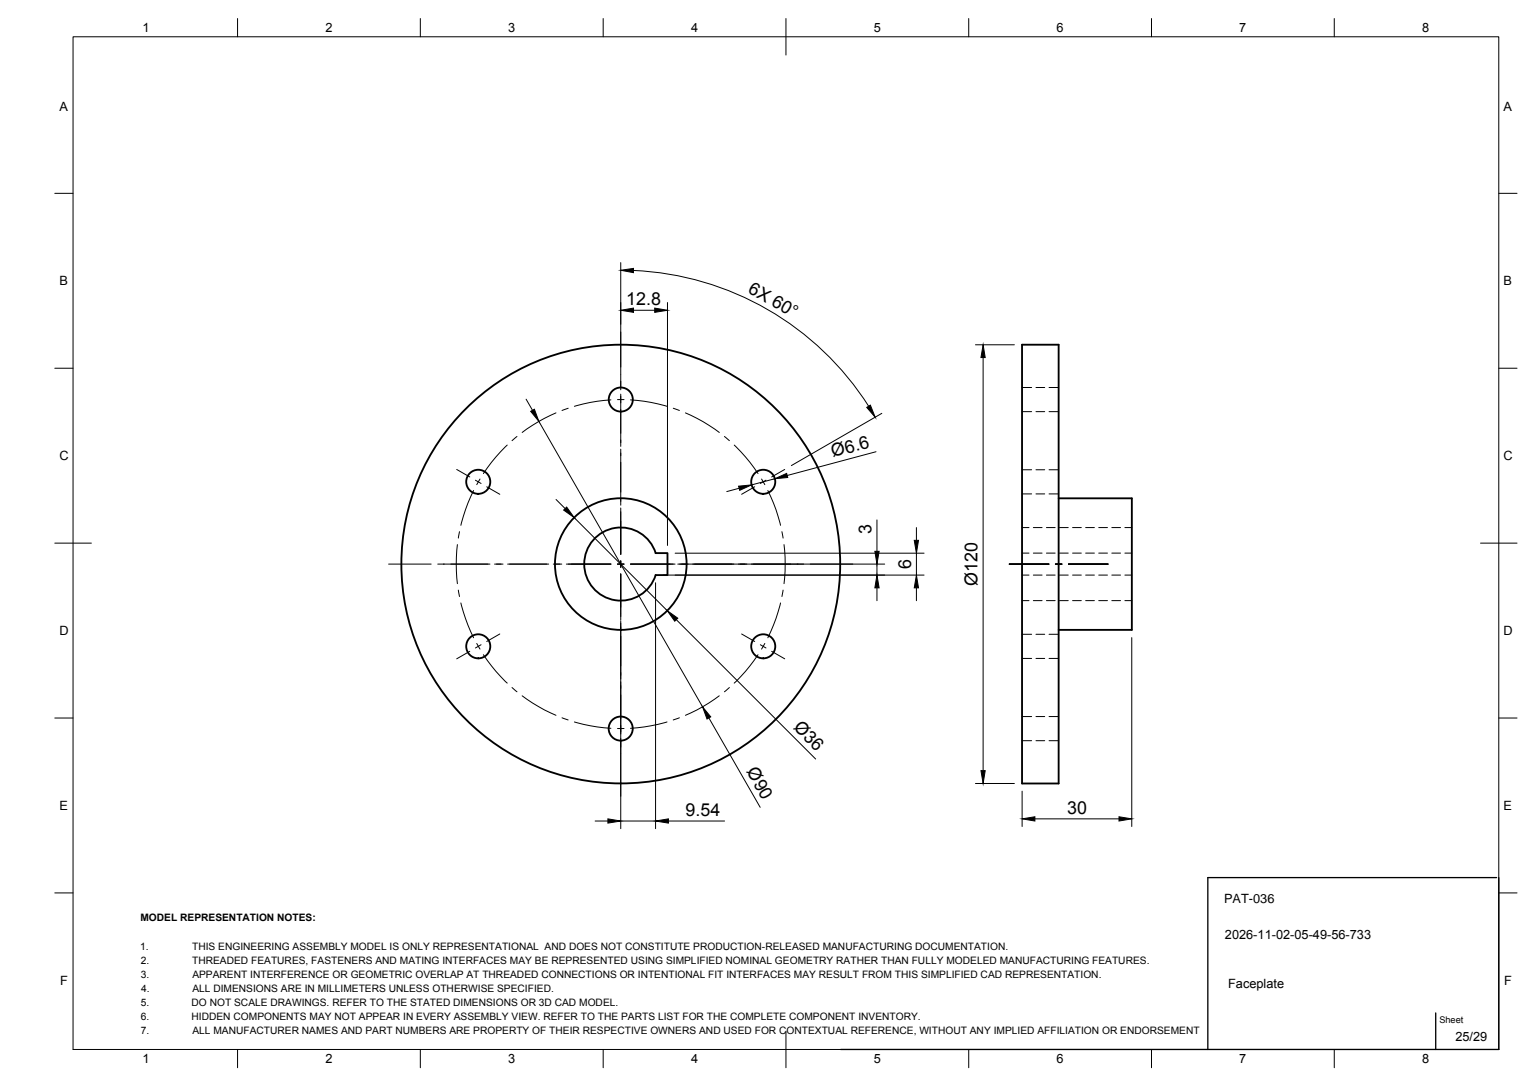
ISO-10303-21;
HEADER;
/* Generated by software containing ST-Developer
 * from STEP Tools, Inc. (www.steptools.com) 
 */

FILE_DESCRIPTION(
/* description */ ('Flange-mounted spindle'),
/* implementation_level */ '2;1');

FILE_NAME(
/* name */ 'Faceplate.step',
/* time_stamp */ '2026-10-27T10:49:51-07:00',
/* author */ (''),
/* organization */ (''),
/* preprocessor_version */ 'ST-DEVELOPER v20.2',
/* originating_system */ 'Autodesk Translation Framework v15.17.0.0',
/* authorisation */ '');

FILE_SCHEMA (('AUTOMOTIVE_DESIGN { 1 0 10303 214 3 1 1 }'));
ENDSEC;

DATA;
#10=MECHANICAL_DESIGN_GEOMETRIC_PRESENTATION_REPRESENTATION('',(#357),#11764);
#302=SHAPE_REPRESENTATION_RELATIONSHIP('SRR','None',#11900,#329);
#329=ADVANCED_BREP_SHAPE_REPRESENTATION('',(#383),#11755);
#357=STYLED_ITEM('',(#12085),#383);
#383=MANIFOLD_SOLID_BREP('Body1',#6151);
#471=FACE_BOUND('',#1269,.T.);
#472=FACE_BOUND('',#1270,.T.);
#473=FACE_BOUND('',#1271,.T.);
#474=FACE_BOUND('',#1272,.T.);
#475=FACE_BOUND('',#1273,.T.);
#476=FACE_BOUND('',#1274,.T.);
#477=FACE_BOUND('',#1275,.T.);
#478=FACE_BOUND('',#1284,.T.);
#479=FACE_BOUND('',#1285,.T.);
#480=FACE_BOUND('',#1286,.T.);
#481=FACE_BOUND('',#1287,.T.);
#482=FACE_BOUND('',#1288,.T.);
#483=FACE_BOUND('',#1289,.T.);
#484=FACE_BOUND('',#1290,.T.);
#485=FACE_BOUND('',#1294,.T.);
#608=PLANE('',#6765);
#609=PLANE('',#6766);
#610=PLANE('',#6767);
#611=PLANE('',#6768);
#612=PLANE('',#6791);
#613=PLANE('',#6797);
#840=FACE_OUTER_BOUND('',#1265,.T.);
#841=FACE_OUTER_BOUND('',#1266,.T.);
#842=FACE_OUTER_BOUND('',#1267,.T.);
#843=FACE_OUTER_BOUND('',#1268,.T.);
#844=FACE_OUTER_BOUND('',#1276,.T.);
#845=FACE_OUTER_BOUND('',#1277,.T.);
#846=FACE_OUTER_BOUND('',#1278,.T.);
#847=FACE_OUTER_BOUND('',#1279,.T.);
#848=FACE_OUTER_BOUND('',#1280,.T.);
#849=FACE_OUTER_BOUND('',#1281,.T.);
#850=FACE_OUTER_BOUND('',#1282,.T.);
#851=FACE_OUTER_BOUND('',#1283,.T.);
#852=FACE_OUTER_BOUND('',#1291,.T.);
#853=FACE_OUTER_BOUND('',#1292,.T.);
#854=FACE_OUTER_BOUND('',#1293,.T.);
#1265=EDGE_LOOP('',(#4699,#4700,#4701,#4702));
#1266=EDGE_LOOP('',(#4703,#4704,#4705,#4706));
#1267=EDGE_LOOP('',(#4707,#4708,#4709,#4710));
#1268=EDGE_LOOP('',(#4711));
#1269=EDGE_LOOP('',(#4712));
#1270=EDGE_LOOP('',(#4713));
#1271=EDGE_LOOP('',(#4714));
#1272=EDGE_LOOP('',(#4715));
#1273=EDGE_LOOP('',(#4716));
#1274=EDGE_LOOP('',(#4717));
#1275=EDGE_LOOP('',(#4718,#4719,#4720,#4721));
#1276=EDGE_LOOP('',(#4722,#4723,#4724,#4725));
#1277=EDGE_LOOP('',(#4726,#4727,#4728,#4729));
#1278=EDGE_LOOP('',(#4730,#4731,#4732,#4733));
#1279=EDGE_LOOP('',(#4734,#4735,#4736,#4737));
#1280=EDGE_LOOP('',(#4738,#4739,#4740,#4741));
#1281=EDGE_LOOP('',(#4742,#4743,#4744,#4745));
#1282=EDGE_LOOP('',(#4746,#4747,#4748,#4749));
#1283=EDGE_LOOP('',(#4750));
#1284=EDGE_LOOP('',(#4751));
#1285=EDGE_LOOP('',(#4752));
#1286=EDGE_LOOP('',(#4753));
#1287=EDGE_LOOP('',(#4754));
#1288=EDGE_LOOP('',(#4755));
#1289=EDGE_LOOP('',(#4756));
#1290=EDGE_LOOP('',(#4757));
#1291=EDGE_LOOP('',(#4758,#4759,#4760,#4761));
#1292=EDGE_LOOP('',(#4762,#4763,#4764,#4765));
#1293=EDGE_LOOP('',(#4766));
#1294=EDGE_LOOP('',(#4767,#4768,#4769,#4770));
#1679=LINE('',#10434,#2101);
#1680=LINE('',#10436,#2102);
#1681=LINE('',#10438,#2103);
#1682=LINE('',#10439,#2104);
#1683=LINE('',#10442,#2105);
#1684=LINE('',#10444,#2106);
#1685=LINE('',#10445,#2107);
#1686=LINE('',#10448,#2108);
#1687=LINE('',#10450,#2109);
#1688=LINE('',#10451,#2110);
#1689=LINE('',#10473,#2111);
#1690=LINE('',#10477,#2112);
#1691=LINE('',#10481,#2113);
#1692=LINE('',#10485,#2114);
#1693=LINE('',#10489,#2115);
#1694=LINE('',#10493,#2116);
#1695=LINE('',#10500,#2117);
#1696=LINE('',#10503,#2118);
#2101=VECTOR('',#8022,1.);
#2102=VECTOR('',#8023,1.);
#2103=VECTOR('',#8024,1.);
#2104=VECTOR('',#8025,1.);
#2105=VECTOR('',#8028,1.);
#2106=VECTOR('',#8029,1.);
#2107=VECTOR('',#8030,1.);
#2108=VECTOR('',#8033,1.);
#2109=VECTOR('',#8034,1.);
#2110=VECTOR('',#8035,1.);
#2111=VECTOR('',#8062,0.33);
#2112=VECTOR('',#8067,0.33);
#2113=VECTOR('',#8072,0.33);
#2114=VECTOR('',#8077,0.33);
#2115=VECTOR('',#8082,0.33);
#2116=VECTOR('',#8087,0.33);
#2117=VECTOR('',#8096,6.);
#2118=VECTOR('',#8099,1.8);
#2438=CIRCLE('',#6769,6.);
#2439=CIRCLE('',#6770,0.33);
#2440=CIRCLE('',#6771,0.33);
#2441=CIRCLE('',#6772,0.33);
#2442=CIRCLE('',#6773,0.33);
#2443=CIRCLE('',#6774,0.33);
#2444=CIRCLE('',#6775,0.33);
#2445=CIRCLE('',#6776,1.);
#2446=CIRCLE('',#6778,1.);
#2447=CIRCLE('',#6780,0.33);
#2448=CIRCLE('',#6782,0.33);
#2449=CIRCLE('',#6784,0.33);
#2450=CIRCLE('',#6786,0.33);
#2451=CIRCLE('',#6788,0.33);
#2452=CIRCLE('',#6790,0.33);
#2453=CIRCLE('',#6792,6.);
#2454=CIRCLE('',#6793,1.8);
#2455=CIRCLE('',#6796,1.8);
#2886=VERTEX_POINT('',#10432);
#2887=VERTEX_POINT('',#10433);
#2888=VERTEX_POINT('',#10435);
#2889=VERTEX_POINT('',#10437);
#2890=VERTEX_POINT('',#10441);
#2891=VERTEX_POINT('',#10443);
#2892=VERTEX_POINT('',#10447);
#2893=VERTEX_POINT('',#10449);
#2894=VERTEX_POINT('',#10453);
#2895=VERTEX_POINT('',#10455);
#2896=VERTEX_POINT('',#10457);
#2897=VERTEX_POINT('',#10459);
#2898=VERTEX_POINT('',#10461);
#2899=VERTEX_POINT('',#10463);
#2900=VERTEX_POINT('',#10465);
#2901=VERTEX_POINT('',#10471);
#2902=VERTEX_POINT('',#10475);
#2903=VERTEX_POINT('',#10479);
#2904=VERTEX_POINT('',#10483);
#2905=VERTEX_POINT('',#10487);
#2906=VERTEX_POINT('',#10491);
#2907=VERTEX_POINT('',#10495);
#2908=VERTEX_POINT('',#10497);
#2909=VERTEX_POINT('',#10502);
#3542=EDGE_CURVE('',#2886,#2887,#1679,.T.);
#3543=EDGE_CURVE('',#2886,#2888,#1680,.T.);
#3544=EDGE_CURVE('',#2889,#2888,#1681,.T.);
#3545=EDGE_CURVE('',#2887,#2889,#1682,.T.);
#3546=EDGE_CURVE('',#2890,#2886,#1683,.T.);
#3547=EDGE_CURVE('',#2890,#2891,#1684,.T.);
#3548=EDGE_CURVE('',#2888,#2891,#1685,.T.);
#3549=EDGE_CURVE('',#2892,#2890,#1686,.T.);
#3550=EDGE_CURVE('',#2893,#2892,#1687,.T.);
#3551=EDGE_CURVE('',#2891,#2893,#1688,.T.);
#3552=EDGE_CURVE('',#2894,#2894,#2438,.T.);
#3553=EDGE_CURVE('',#2895,#2895,#2439,.T.);
#3554=EDGE_CURVE('',#2896,#2896,#2440,.T.);
#3555=EDGE_CURVE('',#2897,#2897,#2441,.T.);
#3556=EDGE_CURVE('',#2898,#2898,#2442,.T.);
#3557=EDGE_CURVE('',#2899,#2899,#2443,.T.);
#3558=EDGE_CURVE('',#2900,#2900,#2444,.T.);
#3559=EDGE_CURVE('',#2893,#2889,#2445,.T.);
#3560=EDGE_CURVE('',#2892,#2887,#2446,.T.);
#3561=EDGE_CURVE('',#2901,#2901,#2447,.T.);
#3562=EDGE_CURVE('',#2901,#2895,#1689,.T.);
#3563=EDGE_CURVE('',#2902,#2902,#2448,.T.);
#3564=EDGE_CURVE('',#2902,#2896,#1690,.T.);
#3565=EDGE_CURVE('',#2903,#2903,#2449,.T.);
#3566=EDGE_CURVE('',#2903,#2897,#1691,.T.);
#3567=EDGE_CURVE('',#2904,#2904,#2450,.T.);
#3568=EDGE_CURVE('',#2904,#2898,#1692,.T.);
#3569=EDGE_CURVE('',#2905,#2905,#2451,.T.);
#3570=EDGE_CURVE('',#2905,#2899,#1693,.T.);
#3571=EDGE_CURVE('',#2906,#2906,#2452,.T.);
#3572=EDGE_CURVE('',#2906,#2900,#1694,.T.);
#3573=EDGE_CURVE('',#2907,#2907,#2453,.T.);
#3574=EDGE_CURVE('',#2908,#2908,#2454,.T.);
#3575=EDGE_CURVE('',#2894,#2907,#1695,.T.);
#3576=EDGE_CURVE('',#2908,#2909,#1696,.T.);
#3577=EDGE_CURVE('',#2909,#2909,#2455,.T.);
#4699=ORIENTED_EDGE('',*,*,#3542,.F.);
#4700=ORIENTED_EDGE('',*,*,#3543,.T.);
#4701=ORIENTED_EDGE('',*,*,#3544,.F.);
#4702=ORIENTED_EDGE('',*,*,#3545,.F.);
#4703=ORIENTED_EDGE('',*,*,#3546,.F.);
#4704=ORIENTED_EDGE('',*,*,#3547,.T.);
#4705=ORIENTED_EDGE('',*,*,#3548,.F.);
#4706=ORIENTED_EDGE('',*,*,#3543,.F.);
#4707=ORIENTED_EDGE('',*,*,#3549,.F.);
#4708=ORIENTED_EDGE('',*,*,#3550,.F.);
#4709=ORIENTED_EDGE('',*,*,#3551,.F.);
#4710=ORIENTED_EDGE('',*,*,#3547,.F.);
#4711=ORIENTED_EDGE('',*,*,#3552,.T.);
#4712=ORIENTED_EDGE('',*,*,#3553,.T.);
#4713=ORIENTED_EDGE('',*,*,#3554,.T.);
#4714=ORIENTED_EDGE('',*,*,#3555,.T.);
#4715=ORIENTED_EDGE('',*,*,#3556,.T.);
#4716=ORIENTED_EDGE('',*,*,#3557,.T.);
#4717=ORIENTED_EDGE('',*,*,#3558,.T.);
#4718=ORIENTED_EDGE('',*,*,#3544,.T.);
#4719=ORIENTED_EDGE('',*,*,#3548,.T.);
#4720=ORIENTED_EDGE('',*,*,#3551,.T.);
#4721=ORIENTED_EDGE('',*,*,#3559,.T.);
#4722=ORIENTED_EDGE('',*,*,#3545,.T.);
#4723=ORIENTED_EDGE('',*,*,#3559,.F.);
#4724=ORIENTED_EDGE('',*,*,#3550,.T.);
#4725=ORIENTED_EDGE('',*,*,#3560,.T.);
#4726=ORIENTED_EDGE('',*,*,#3561,.F.);
#4727=ORIENTED_EDGE('',*,*,#3562,.T.);
#4728=ORIENTED_EDGE('',*,*,#3553,.F.);
#4729=ORIENTED_EDGE('',*,*,#3562,.F.);
#4730=ORIENTED_EDGE('',*,*,#3563,.F.);
#4731=ORIENTED_EDGE('',*,*,#3564,.T.);
#4732=ORIENTED_EDGE('',*,*,#3554,.F.);
#4733=ORIENTED_EDGE('',*,*,#3564,.F.);
#4734=ORIENTED_EDGE('',*,*,#3565,.F.);
#4735=ORIENTED_EDGE('',*,*,#3566,.T.);
#4736=ORIENTED_EDGE('',*,*,#3555,.F.);
#4737=ORIENTED_EDGE('',*,*,#3566,.F.);
#4738=ORIENTED_EDGE('',*,*,#3567,.F.);
#4739=ORIENTED_EDGE('',*,*,#3568,.T.);
#4740=ORIENTED_EDGE('',*,*,#3556,.F.);
#4741=ORIENTED_EDGE('',*,*,#3568,.F.);
#4742=ORIENTED_EDGE('',*,*,#3569,.F.);
#4743=ORIENTED_EDGE('',*,*,#3570,.T.);
#4744=ORIENTED_EDGE('',*,*,#3557,.F.);
#4745=ORIENTED_EDGE('',*,*,#3570,.F.);
#4746=ORIENTED_EDGE('',*,*,#3571,.F.);
#4747=ORIENTED_EDGE('',*,*,#3572,.T.);
#4748=ORIENTED_EDGE('',*,*,#3558,.F.);
#4749=ORIENTED_EDGE('',*,*,#3572,.F.);
#4750=ORIENTED_EDGE('',*,*,#3573,.F.);
#4751=ORIENTED_EDGE('',*,*,#3574,.F.);
#4752=ORIENTED_EDGE('',*,*,#3571,.T.);
#4753=ORIENTED_EDGE('',*,*,#3569,.T.);
#4754=ORIENTED_EDGE('',*,*,#3567,.T.);
#4755=ORIENTED_EDGE('',*,*,#3565,.T.);
#4756=ORIENTED_EDGE('',*,*,#3563,.T.);
#4757=ORIENTED_EDGE('',*,*,#3561,.T.);
#4758=ORIENTED_EDGE('',*,*,#3552,.F.);
#4759=ORIENTED_EDGE('',*,*,#3575,.T.);
#4760=ORIENTED_EDGE('',*,*,#3573,.T.);
#4761=ORIENTED_EDGE('',*,*,#3575,.F.);
#4762=ORIENTED_EDGE('',*,*,#3574,.T.);
#4763=ORIENTED_EDGE('',*,*,#3576,.T.);
#4764=ORIENTED_EDGE('',*,*,#3577,.T.);
#4765=ORIENTED_EDGE('',*,*,#3576,.F.);
#4766=ORIENTED_EDGE('',*,*,#3577,.F.);
#4767=ORIENTED_EDGE('',*,*,#3542,.T.);
#4768=ORIENTED_EDGE('',*,*,#3560,.F.);
#4769=ORIENTED_EDGE('',*,*,#3549,.T.);
#4770=ORIENTED_EDGE('',*,*,#3546,.T.);
#5680=CYLINDRICAL_SURFACE('',#6777,1.);
#5681=CYLINDRICAL_SURFACE('',#6779,0.33);
#5682=CYLINDRICAL_SURFACE('',#6781,0.33);
#5683=CYLINDRICAL_SURFACE('',#6783,0.33);
#5684=CYLINDRICAL_SURFACE('',#6785,0.33);
#5685=CYLINDRICAL_SURFACE('',#6787,0.33);
#5686=CYLINDRICAL_SURFACE('',#6789,0.33);
#5687=CYLINDRICAL_SURFACE('',#6794,6.);
#5688=CYLINDRICAL_SURFACE('',#6795,1.8);
#5951=ADVANCED_FACE('',(#840),#608,.F.);
#5952=ADVANCED_FACE('',(#841),#609,.F.);
#5953=ADVANCED_FACE('',(#842),#610,.F.);
#5954=ADVANCED_FACE('',(#843,#471,#472,#473,#474,#475,#476,#477),#611,.T.);
#5955=ADVANCED_FACE('',(#844),#5680,.F.);
#5956=ADVANCED_FACE('',(#845),#5681,.F.);
#5957=ADVANCED_FACE('',(#846),#5682,.F.);
#5958=ADVANCED_FACE('',(#847),#5683,.F.);
#5959=ADVANCED_FACE('',(#848),#5684,.F.);
#5960=ADVANCED_FACE('',(#849),#5685,.F.);
#5961=ADVANCED_FACE('',(#850),#5686,.F.);
#5962=ADVANCED_FACE('',(#851,#478,#479,#480,#481,#482,#483,#484),#612,.F.);
#5963=ADVANCED_FACE('',(#852),#5687,.T.);
#5964=ADVANCED_FACE('',(#853),#5688,.T.);
#5965=ADVANCED_FACE('',(#854,#485),#613,.F.);
#6151=CLOSED_SHELL('',(#5951,#5952,#5953,#5954,#5955,#5956,#5957,#5958,
#5959,#5960,#5961,#5962,#5963,#5964,#5965));
#6764=AXIS2_PLACEMENT_3D('',#10430,#8018,#8019);
#6765=AXIS2_PLACEMENT_3D('',#10431,#8020,#8021);
#6766=AXIS2_PLACEMENT_3D('',#10440,#8026,#8027);
#6767=AXIS2_PLACEMENT_3D('',#10446,#8031,#8032);
#6768=AXIS2_PLACEMENT_3D('',#10452,#8036,#8037);
#6769=AXIS2_PLACEMENT_3D('',#10454,#8038,#8039);
#6770=AXIS2_PLACEMENT_3D('',#10456,#8040,#8041);
#6771=AXIS2_PLACEMENT_3D('',#10458,#8042,#8043);
#6772=AXIS2_PLACEMENT_3D('',#10460,#8044,#8045);
#6773=AXIS2_PLACEMENT_3D('',#10462,#8046,#8047);
#6774=AXIS2_PLACEMENT_3D('',#10464,#8048,#8049);
#6775=AXIS2_PLACEMENT_3D('',#10466,#8050,#8051);
#6776=AXIS2_PLACEMENT_3D('',#10467,#8052,#8053);
#6777=AXIS2_PLACEMENT_3D('',#10468,#8054,#8055);
#6778=AXIS2_PLACEMENT_3D('',#10469,#8056,#8057);
#6779=AXIS2_PLACEMENT_3D('',#10470,#8058,#8059);
#6780=AXIS2_PLACEMENT_3D('',#10472,#8060,#8061);
#6781=AXIS2_PLACEMENT_3D('',#10474,#8063,#8064);
#6782=AXIS2_PLACEMENT_3D('',#10476,#8065,#8066);
#6783=AXIS2_PLACEMENT_3D('',#10478,#8068,#8069);
#6784=AXIS2_PLACEMENT_3D('',#10480,#8070,#8071);
#6785=AXIS2_PLACEMENT_3D('',#10482,#8073,#8074);
#6786=AXIS2_PLACEMENT_3D('',#10484,#8075,#8076);
#6787=AXIS2_PLACEMENT_3D('',#10486,#8078,#8079);
#6788=AXIS2_PLACEMENT_3D('',#10488,#8080,#8081);
#6789=AXIS2_PLACEMENT_3D('',#10490,#8083,#8084);
#6790=AXIS2_PLACEMENT_3D('',#10492,#8085,#8086);
#6791=AXIS2_PLACEMENT_3D('',#10494,#8088,#8089);
#6792=AXIS2_PLACEMENT_3D('',#10496,#8090,#8091);
#6793=AXIS2_PLACEMENT_3D('',#10498,#8092,#8093);
#6794=AXIS2_PLACEMENT_3D('',#10499,#8094,#8095);
#6795=AXIS2_PLACEMENT_3D('',#10501,#8097,#8098);
#6796=AXIS2_PLACEMENT_3D('',#10504,#8100,#8101);
#6797=AXIS2_PLACEMENT_3D('',#10505,#8102,#8103);
#8018=DIRECTION('axis',(0.,0.,1.));
#8019=DIRECTION('refdir',(1.,0.,0.));
#8020=DIRECTION('center_axis',(-1.,0.,0.));
#8021=DIRECTION('ref_axis',(0.,0.,1.));
#8022=DIRECTION('',(0.,0.,1.));
#8023=DIRECTION('',(0.,1.,0.));
#8024=DIRECTION('',(0.,0.,-1.));
#8025=DIRECTION('',(0.,1.,0.));
#8026=DIRECTION('center_axis',(0.,0.,-1.));
#8027=DIRECTION('ref_axis',(-1.,0.,0.));
#8028=DIRECTION('',(-1.,0.,0.));
#8029=DIRECTION('',(0.,1.,0.));
#8030=DIRECTION('',(1.,0.,0.));
#8031=DIRECTION('center_axis',(1.,0.,0.));
#8032=DIRECTION('ref_axis',(0.,0.,-1.));
#8033=DIRECTION('',(0.,0.,-1.));
#8034=DIRECTION('',(0.,-1.,0.));
#8035=DIRECTION('',(0.,0.,1.));
#8036=DIRECTION('center_axis',(0.,1.,0.));
#8037=DIRECTION('ref_axis',(1.,0.,0.));
#8038=DIRECTION('center_axis',(0.,1.,0.));
#8039=DIRECTION('ref_axis',(1.,0.,0.));
#8040=DIRECTION('center_axis',(0.,-1.,0.));
#8041=DIRECTION('ref_axis',(1.,0.,0.));
#8042=DIRECTION('center_axis',(0.,-1.,0.));
#8043=DIRECTION('ref_axis',(1.,0.,0.));
#8044=DIRECTION('center_axis',(0.,-1.,0.));
#8045=DIRECTION('ref_axis',(1.,0.,0.));
#8046=DIRECTION('center_axis',(0.,-1.,0.));
#8047=DIRECTION('ref_axis',(1.,0.,0.));
#8048=DIRECTION('center_axis',(0.,-1.,0.));
#8049=DIRECTION('ref_axis',(1.,0.,0.));
#8050=DIRECTION('center_axis',(0.,-1.,0.));
#8051=DIRECTION('ref_axis',(1.,0.,0.));
#8052=DIRECTION('center_axis',(0.,-1.,0.));
#8053=DIRECTION('ref_axis',(1.,0.,0.));
#8054=DIRECTION('center_axis',(0.,1.,0.));
#8055=DIRECTION('ref_axis',(-1.83697019872103E-16,0.,1.));
#8056=DIRECTION('center_axis',(0.,-1.,0.));
#8057=DIRECTION('ref_axis',(1.,0.,0.));
#8058=DIRECTION('center_axis',(0.,1.,0.));
#8059=DIRECTION('ref_axis',(1.,0.,0.));
#8060=DIRECTION('center_axis',(0.,1.,0.));
#8061=DIRECTION('ref_axis',(1.,0.,0.));
#8062=DIRECTION('',(0.,1.,0.));
#8063=DIRECTION('center_axis',(0.,1.,0.));
#8064=DIRECTION('ref_axis',(1.,0.,0.));
#8065=DIRECTION('center_axis',(0.,1.,0.));
#8066=DIRECTION('ref_axis',(1.,0.,0.));
#8067=DIRECTION('',(0.,1.,0.));
#8068=DIRECTION('center_axis',(0.,1.,0.));
#8069=DIRECTION('ref_axis',(1.,0.,0.));
#8070=DIRECTION('center_axis',(0.,1.,0.));
#8071=DIRECTION('ref_axis',(1.,0.,0.));
#8072=DIRECTION('',(0.,1.,0.));
#8073=DIRECTION('center_axis',(0.,1.,0.));
#8074=DIRECTION('ref_axis',(1.,0.,0.));
#8075=DIRECTION('center_axis',(0.,1.,0.));
#8076=DIRECTION('ref_axis',(1.,0.,0.));
#8077=DIRECTION('',(0.,1.,0.));
#8078=DIRECTION('center_axis',(0.,1.,0.));
#8079=DIRECTION('ref_axis',(1.,0.,0.));
#8080=DIRECTION('center_axis',(0.,1.,0.));
#8081=DIRECTION('ref_axis',(1.,0.,0.));
#8082=DIRECTION('',(0.,1.,0.));
#8083=DIRECTION('center_axis',(0.,1.,0.));
#8084=DIRECTION('ref_axis',(1.,0.,0.));
#8085=DIRECTION('center_axis',(0.,1.,0.));
#8086=DIRECTION('ref_axis',(1.,0.,0.));
#8087=DIRECTION('',(0.,1.,0.));
#8088=DIRECTION('center_axis',(0.,1.,0.));
#8089=DIRECTION('ref_axis',(1.,0.,0.));
#8090=DIRECTION('center_axis',(0.,1.,0.));
#8091=DIRECTION('ref_axis',(1.,0.,0.));
#8092=DIRECTION('center_axis',(0.,-1.,0.));
#8093=DIRECTION('ref_axis',(1.,0.,0.));
#8094=DIRECTION('center_axis',(0.,1.,0.));
#8095=DIRECTION('ref_axis',(1.,0.,0.));
#8096=DIRECTION('',(0.,-1.,0.));
#8097=DIRECTION('center_axis',(0.,1.,0.));
#8098=DIRECTION('ref_axis',(1.,0.,0.));
#8099=DIRECTION('',(0.,-1.,0.));
#8100=DIRECTION('center_axis',(0.,1.,0.));
#8101=DIRECTION('ref_axis',(1.,0.,0.));
#8102=DIRECTION('center_axis',(0.,1.,0.));
#8103=DIRECTION('ref_axis',(1.,0.,0.));
#10430=CARTESIAN_POINT('',(0.,0.,0.));
#10431=CARTESIAN_POINT('Origin',(-0.3,3.4,6.72));
#10432=CARTESIAN_POINT('',(-0.3,3.5,6.72));
#10433=CARTESIAN_POINT('',(-0.3,3.5,7.04606079858305));
#10434=CARTESIAN_POINT('',(-0.3,3.5,7.36));
#10435=CARTESIAN_POINT('',(-0.3,6.5,6.72));
#10436=CARTESIAN_POINT('',(-0.3,3.4,6.72));
#10437=CARTESIAN_POINT('',(-0.3,6.5,7.04606079858305));
#10438=CARTESIAN_POINT('',(-0.3,6.5,7.36));
#10439=CARTESIAN_POINT('',(-0.3,3.5,7.04606079858305));
#10440=CARTESIAN_POINT('Origin',(0.3,3.4,6.72));
#10441=CARTESIAN_POINT('',(0.3,3.5,6.72));
#10442=CARTESIAN_POINT('',(0.15,3.5,6.72));
#10443=CARTESIAN_POINT('',(0.3,6.5,6.72));
#10444=CARTESIAN_POINT('',(0.3,3.4,6.72));
#10445=CARTESIAN_POINT('',(0.15,6.5,6.72));
#10446=CARTESIAN_POINT('Origin',(0.3,3.4,8.));
#10447=CARTESIAN_POINT('',(0.3,3.5,7.04606079858305));
#10448=CARTESIAN_POINT('',(0.3,3.5,8.));
#10449=CARTESIAN_POINT('',(0.3,6.5,7.04606079858305));
#10450=CARTESIAN_POINT('',(0.3,3.5,7.04606079858305));
#10451=CARTESIAN_POINT('',(0.3,6.5,8.));
#10452=CARTESIAN_POINT('Origin',(0.,6.5,8.));
#10453=CARTESIAN_POINT('',(-6.,6.5,8.));
#10454=CARTESIAN_POINT('Origin',(0.,6.5,8.));
#10455=CARTESIAN_POINT('',(-2.58,6.5,4.10288568297003));
#10456=CARTESIAN_POINT('Origin',(-2.25,6.5,4.10288568297003));
#10457=CARTESIAN_POINT('',(4.17,6.5,8.));
#10458=CARTESIAN_POINT('Origin',(4.5,6.5,8.));
#10459=CARTESIAN_POINT('',(1.92,6.5,11.89711431703));
#10460=CARTESIAN_POINT('Origin',(2.25,6.5,11.89711431703));
#10461=CARTESIAN_POINT('',(-2.58,6.5,11.89711431703));
#10462=CARTESIAN_POINT('Origin',(-2.25,6.5,11.89711431703));
#10463=CARTESIAN_POINT('',(-4.83,6.5,8.));
#10464=CARTESIAN_POINT('Origin',(-4.5,6.5,8.));
#10465=CARTESIAN_POINT('',(1.92,6.5,4.10288568297003));
#10466=CARTESIAN_POINT('Origin',(2.25,6.5,4.10288568297003));
#10467=CARTESIAN_POINT('Origin',(0.,6.5,8.));
#10468=CARTESIAN_POINT('Origin',(0.,3.5,8.));
#10469=CARTESIAN_POINT('Origin',(0.,3.5,8.));
#10470=CARTESIAN_POINT('Origin',(-2.25,5.4,4.10288568297003));
#10471=CARTESIAN_POINT('',(-2.58,5.5,4.10288568297003));
#10472=CARTESIAN_POINT('Origin',(-2.25,5.5,4.10288568297003));
#10473=CARTESIAN_POINT('',(-2.58,5.4,4.10288568297003));
#10474=CARTESIAN_POINT('Origin',(4.5,5.4,8.));
#10475=CARTESIAN_POINT('',(4.17,5.5,8.));
#10476=CARTESIAN_POINT('Origin',(4.5,5.5,8.));
#10477=CARTESIAN_POINT('',(4.17,5.4,8.));
#10478=CARTESIAN_POINT('Origin',(2.25,5.4,11.89711431703));
#10479=CARTESIAN_POINT('',(1.92,5.5,11.89711431703));
#10480=CARTESIAN_POINT('Origin',(2.25,5.5,11.89711431703));
#10481=CARTESIAN_POINT('',(1.92,5.4,11.89711431703));
#10482=CARTESIAN_POINT('Origin',(-2.25,5.4,11.89711431703));
#10483=CARTESIAN_POINT('',(-2.58,5.5,11.89711431703));
#10484=CARTESIAN_POINT('Origin',(-2.25,5.5,11.89711431703));
#10485=CARTESIAN_POINT('',(-2.58,5.4,11.89711431703));
#10486=CARTESIAN_POINT('Origin',(-4.5,5.4,8.));
#10487=CARTESIAN_POINT('',(-4.83,5.5,8.));
#10488=CARTESIAN_POINT('Origin',(-4.5,5.5,8.));
#10489=CARTESIAN_POINT('',(-4.83,5.4,8.));
#10490=CARTESIAN_POINT('Origin',(2.25,5.4,4.10288568297003));
#10491=CARTESIAN_POINT('',(1.92,5.5,4.10288568297003));
#10492=CARTESIAN_POINT('Origin',(2.25,5.5,4.10288568297003));
#10493=CARTESIAN_POINT('',(1.92,5.4,4.10288568297003));
#10494=CARTESIAN_POINT('Origin',(0.,5.5,8.));
#10495=CARTESIAN_POINT('',(-6.,5.5,8.));
#10496=CARTESIAN_POINT('Origin',(0.,5.5,8.));
#10497=CARTESIAN_POINT('',(-1.8,5.5,8.));
#10498=CARTESIAN_POINT('Origin',(0.,5.5,8.));
#10499=CARTESIAN_POINT('Origin',(0.,5.5,8.));
#10500=CARTESIAN_POINT('',(-6.,5.5,8.));
#10501=CARTESIAN_POINT('Origin',(0.,3.5,8.));
#10502=CARTESIAN_POINT('',(-1.8,3.5,8.));
#10503=CARTESIAN_POINT('',(-1.8,3.5,8.));
#10504=CARTESIAN_POINT('Origin',(0.,3.5,8.));
#10505=CARTESIAN_POINT('Origin',(0.,3.5,8.));
#11723=UNCERTAINTY_MEASURE_WITH_UNIT(LENGTH_MEASURE(0.001),#11765,
'DISTANCE_ACCURACY_VALUE',
'Maximum model space distance between geometric entities at asserted c
onnectivities');
#11732=UNCERTAINTY_MEASURE_WITH_UNIT(LENGTH_MEASURE(0.001),#11765,
'DISTANCE_ACCURACY_VALUE',
'Maximum model space distance between geometric entities at asserted c
onnectivities');
#11755=(
GEOMETRIC_REPRESENTATION_CONTEXT(3)
GLOBAL_UNCERTAINTY_ASSIGNED_CONTEXT((#11723))
GLOBAL_UNIT_ASSIGNED_CONTEXT((#11765,#11767,#11768))
REPRESENTATION_CONTEXT('','3D')
);
#11764=(
GEOMETRIC_REPRESENTATION_CONTEXT(3)
GLOBAL_UNCERTAINTY_ASSIGNED_CONTEXT((#11732))
GLOBAL_UNIT_ASSIGNED_CONTEXT((#11765,#11767,#11768))
REPRESENTATION_CONTEXT('','3D')
);
#11765=(
LENGTH_UNIT()
NAMED_UNIT(*)
SI_UNIT(.CENTI.,.METRE.)
);
#11767=(
NAMED_UNIT(*)
PLANE_ANGLE_UNIT()
SI_UNIT($,.RADIAN.)
);
#11768=(
NAMED_UNIT(*)
SI_UNIT($,.STERADIAN.)
SOLID_ANGLE_UNIT()
);
#11791=SHAPE_DEFINITION_REPRESENTATION(#11824,#11900);
#11824=PRODUCT_DEFINITION_SHAPE('',$,#11932);
#11900=SHAPE_REPRESENTATION('',(#6764),#11755);
#11909=PRODUCT_DEFINITION_CONTEXT('part definition',#12004,'design');
#11932=PRODUCT_DEFINITION('Faceplate','Faceplate',#11963,#11909);
#11963=PRODUCT_DEFINITION_FORMATION('',$,#12028);
#12004=APPLICATION_CONTEXT(
'Core Data for Automotive Mechanical Design Process');
#12005=PRODUCT_CONTEXT('part definition',#12004,'mechanical');
#12028=PRODUCT('Faceplate','Faceplate','Faceplate',(#12005));
#12079=COLOUR_RGB('Light Blue',0.38,0.62,0.78);
#12080=FILL_AREA_STYLE_COLOUR('',#12079);
#12081=FILL_AREA_STYLE('',(#12080));
#12082=SURFACE_STYLE_FILL_AREA(#12081);
#12083=SURFACE_SIDE_STYLE('',(#12082));
#12084=SURFACE_STYLE_USAGE(.BOTH.,#12083);
#12085=PRESENTATION_STYLE_ASSIGNMENT((#12084));
ENDSEC;
END-ISO-10303-21;
